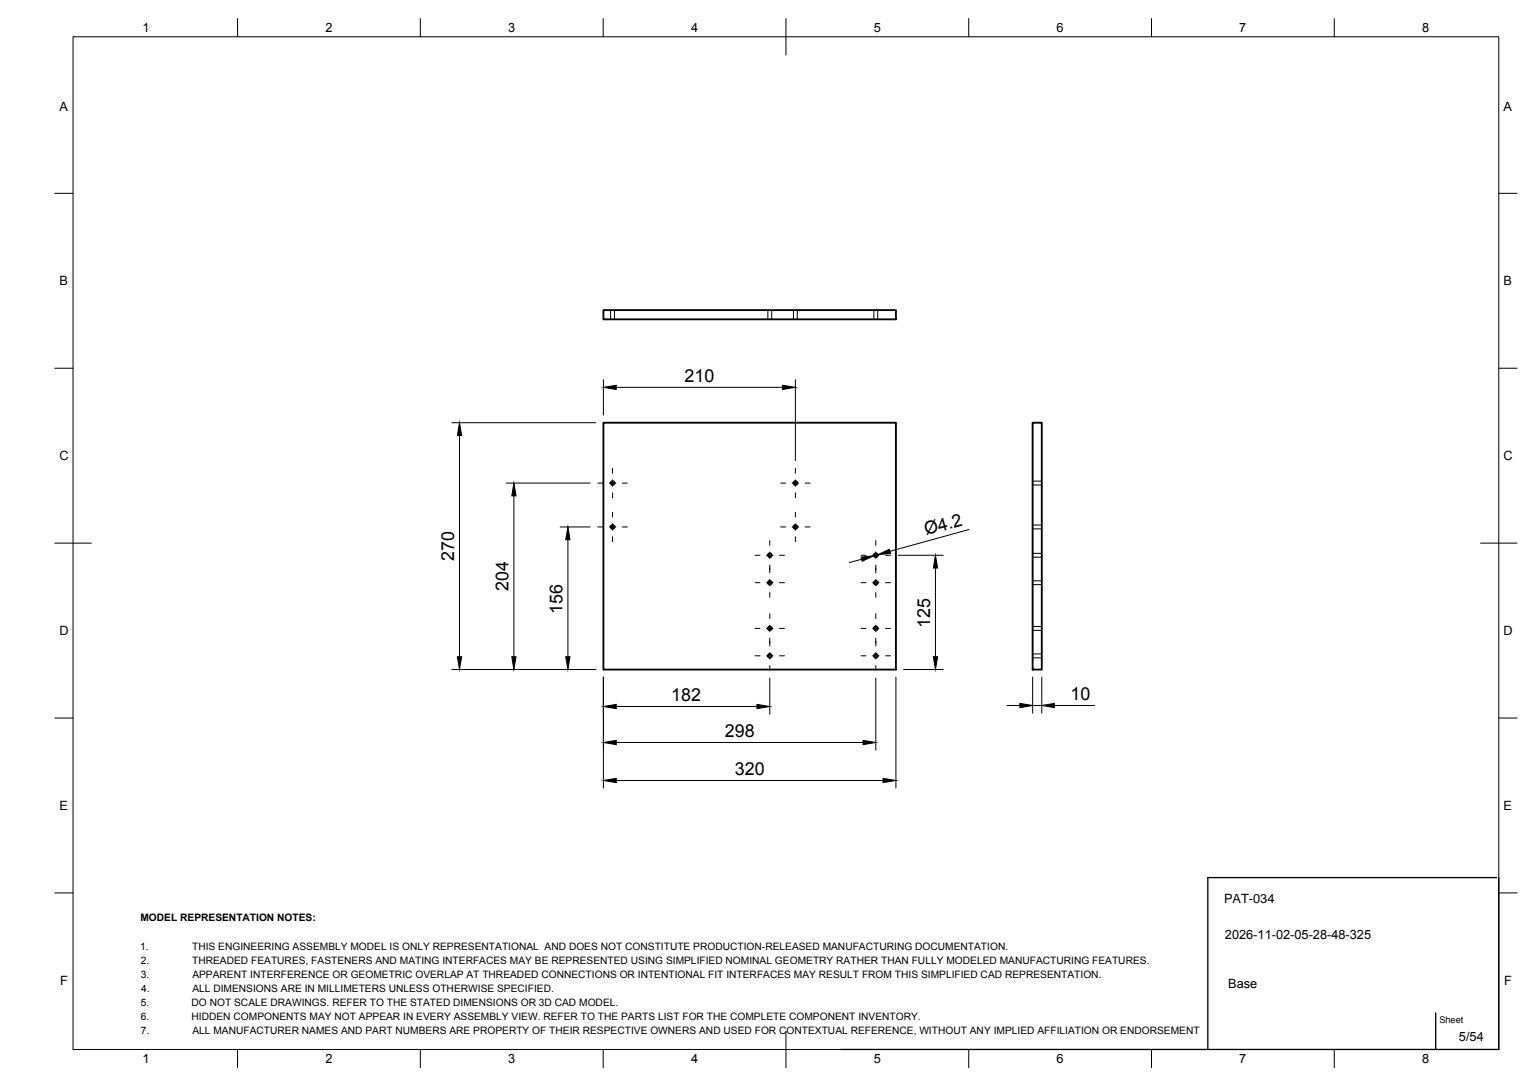
ISO-10303-21;
HEADER;
/* Generated by software containing ST-Developer
 * from STEP Tools, Inc. (www.steptools.com) 
 */

FILE_DESCRIPTION(
/* description */ ('Fatigue rig crank-slider'),
/* implementation_level */ '2;1');

FILE_NAME(
/* name */ 'Base.step',
/* time_stamp */ '2026-10-28T03:24:50-07:00',
/* author */ (''),
/* organization */ (''),
/* preprocessor_version */ 'ST-DEVELOPER v20.2',
/* originating_system */ 'Autodesk Translation Framework v15.17.0.0',
/* authorisation */ '');

FILE_SCHEMA (('AUTOMOTIVE_DESIGN { 1 0 10303 214 3 1 1 }'));
ENDSEC;

DATA;
#10=MECHANICAL_DESIGN_GEOMETRIC_PRESENTATION_REPRESENTATION('',(#587),#16911);
#487=SHAPE_REPRESENTATION_RELATIONSHIP('SRR','None',#17126,#537);
#537=ADVANCED_BREP_SHAPE_REPRESENTATION('',(#646),#16855);
#587=STYLED_ITEM('',(#17466),#646);
#646=MANIFOLD_SOLID_BREP('Body1',#8878);
#700=FACE_BOUND('',#1757,.T.);
#701=FACE_BOUND('',#1758,.T.);
#702=FACE_BOUND('',#1759,.T.);
#703=FACE_BOUND('',#1760,.T.);
#704=FACE_BOUND('',#1761,.T.);
#705=FACE_BOUND('',#1762,.T.);
#706=FACE_BOUND('',#1763,.T.);
#707=FACE_BOUND('',#1764,.T.);
#708=FACE_BOUND('',#1765,.T.);
#709=FACE_BOUND('',#1766,.T.);
#710=FACE_BOUND('',#1767,.T.);
#711=FACE_BOUND('',#1768,.T.);
#712=FACE_BOUND('',#1770,.T.);
#713=FACE_BOUND('',#1771,.T.);
#714=FACE_BOUND('',#1772,.T.);
#715=FACE_BOUND('',#1773,.T.);
#716=FACE_BOUND('',#1774,.T.);
#717=FACE_BOUND('',#1775,.T.);
#718=FACE_BOUND('',#1776,.T.);
#719=FACE_BOUND('',#1777,.T.);
#720=FACE_BOUND('',#1778,.T.);
#721=FACE_BOUND('',#1779,.T.);
#722=FACE_BOUND('',#1780,.T.);
#723=FACE_BOUND('',#1781,.T.);
#897=PLANE('',#9532);
#898=PLANE('',#9533);
#899=PLANE('',#9534);
#900=PLANE('',#9535);
#901=PLANE('',#9536);
#902=PLANE('',#9537);
#1217=FACE_OUTER_BOUND('',#1740,.T.);
#1218=FACE_OUTER_BOUND('',#1741,.T.);
#1219=FACE_OUTER_BOUND('',#1742,.T.);
#1220=FACE_OUTER_BOUND('',#1743,.T.);
#1221=FACE_OUTER_BOUND('',#1744,.T.);
#1222=FACE_OUTER_BOUND('',#1745,.T.);
#1223=FACE_OUTER_BOUND('',#1746,.T.);
#1224=FACE_OUTER_BOUND('',#1747,.T.);
#1225=FACE_OUTER_BOUND('',#1748,.T.);
#1226=FACE_OUTER_BOUND('',#1749,.T.);
#1227=FACE_OUTER_BOUND('',#1750,.T.);
#1228=FACE_OUTER_BOUND('',#1751,.T.);
#1229=FACE_OUTER_BOUND('',#1752,.T.);
#1230=FACE_OUTER_BOUND('',#1753,.T.);
#1231=FACE_OUTER_BOUND('',#1754,.T.);
#1232=FACE_OUTER_BOUND('',#1755,.T.);
#1233=FACE_OUTER_BOUND('',#1756,.T.);
#1234=FACE_OUTER_BOUND('',#1769,.T.);
#1740=EDGE_LOOP('',(#5996,#5997,#5998,#5999));
#1741=EDGE_LOOP('',(#6000,#6001,#6002,#6003));
#1742=EDGE_LOOP('',(#6004,#6005,#6006,#6007));
#1743=EDGE_LOOP('',(#6008,#6009,#6010,#6011));
#1744=EDGE_LOOP('',(#6012,#6013,#6014,#6015));
#1745=EDGE_LOOP('',(#6016,#6017,#6018,#6019));
#1746=EDGE_LOOP('',(#6020,#6021,#6022,#6023));
#1747=EDGE_LOOP('',(#6024,#6025,#6026,#6027));
#1748=EDGE_LOOP('',(#6028,#6029,#6030,#6031));
#1749=EDGE_LOOP('',(#6032,#6033,#6034,#6035));
#1750=EDGE_LOOP('',(#6036,#6037,#6038,#6039));
#1751=EDGE_LOOP('',(#6040,#6041,#6042,#6043));
#1752=EDGE_LOOP('',(#6044,#6045,#6046,#6047));
#1753=EDGE_LOOP('',(#6048,#6049,#6050,#6051));
#1754=EDGE_LOOP('',(#6052,#6053,#6054,#6055));
#1755=EDGE_LOOP('',(#6056,#6057,#6058,#6059));
#1756=EDGE_LOOP('',(#6060,#6061,#6062,#6063));
#1757=EDGE_LOOP('',(#6064));
#1758=EDGE_LOOP('',(#6065));
#1759=EDGE_LOOP('',(#6066));
#1760=EDGE_LOOP('',(#6067));
#1761=EDGE_LOOP('',(#6068));
#1762=EDGE_LOOP('',(#6069));
#1763=EDGE_LOOP('',(#6070));
#1764=EDGE_LOOP('',(#6071));
#1765=EDGE_LOOP('',(#6072));
#1766=EDGE_LOOP('',(#6073));
#1767=EDGE_LOOP('',(#6074));
#1768=EDGE_LOOP('',(#6075));
#1769=EDGE_LOOP('',(#6076,#6077,#6078,#6079));
#1770=EDGE_LOOP('',(#6080));
#1771=EDGE_LOOP('',(#6081));
#1772=EDGE_LOOP('',(#6082));
#1773=EDGE_LOOP('',(#6083));
#1774=EDGE_LOOP('',(#6084));
#1775=EDGE_LOOP('',(#6085));
#1776=EDGE_LOOP('',(#6086));
#1777=EDGE_LOOP('',(#6087));
#1778=EDGE_LOOP('',(#6088));
#1779=EDGE_LOOP('',(#6089));
#1780=EDGE_LOOP('',(#6090));
#1781=EDGE_LOOP('',(#6091));
#2460=LINE('',#13365,#3106);
#2461=LINE('',#13371,#3107);
#2462=LINE('',#13377,#3108);
#2463=LINE('',#13383,#3109);
#2464=LINE('',#13389,#3110);
#2465=LINE('',#13395,#3111);
#2466=LINE('',#13401,#3112);
#2467=LINE('',#13407,#3113);
#2468=LINE('',#13413,#3114);
#2469=LINE('',#13419,#3115);
#2470=LINE('',#13425,#3116);
#2471=LINE('',#13431,#3117);
#2472=LINE('',#13436,#3118);
#2473=LINE('',#13438,#3119);
#2474=LINE('',#13440,#3120);
#2475=LINE('',#13441,#3121);
#2476=LINE('',#13444,#3122);
#2477=LINE('',#13446,#3123);
#2478=LINE('',#13447,#3124);
#2479=LINE('',#13450,#3125);
#2480=LINE('',#13452,#3126);
#2481=LINE('',#13453,#3127);
#2482=LINE('',#13455,#3128);
#2483=LINE('',#13456,#3129);
#3106=VECTOR('',#10576,0.210000000000001);
#3107=VECTOR('',#10583,0.21);
#3108=VECTOR('',#10590,0.21);
#3109=VECTOR('',#10597,0.210000000000001);
#3110=VECTOR('',#10604,0.21);
#3111=VECTOR('',#10611,0.21);
#3112=VECTOR('',#10618,0.21);
#3113=VECTOR('',#10625,0.21);
#3114=VECTOR('',#10632,0.21);
#3115=VECTOR('',#10639,0.21);
#3116=VECTOR('',#10646,0.21);
#3117=VECTOR('',#10653,0.21);
#3118=VECTOR('',#10658,1.);
#3119=VECTOR('',#10659,1.);
#3120=VECTOR('',#10660,1.);
#3121=VECTOR('',#10661,1.);
#3122=VECTOR('',#10664,1.);
#3123=VECTOR('',#10665,1.);
#3124=VECTOR('',#10666,1.);
#3125=VECTOR('',#10669,1.);
#3126=VECTOR('',#10670,1.);
#3127=VECTOR('',#10671,1.);
#3128=VECTOR('',#10674,1.);
#3129=VECTOR('',#10675,1.);
#3752=CIRCLE('',#9497,0.210000000000001);
#3753=CIRCLE('',#9498,0.210000000000001);
#3754=CIRCLE('',#9500,0.21);
#3755=CIRCLE('',#9501,0.21);
#3756=CIRCLE('',#9503,0.21);
#3757=CIRCLE('',#9504,0.21);
#3758=CIRCLE('',#9506,0.210000000000001);
#3759=CIRCLE('',#9507,0.210000000000001);
#3760=CIRCLE('',#9509,0.21);
#3761=CIRCLE('',#9510,0.21);
#3762=CIRCLE('',#9512,0.21);
#3763=CIRCLE('',#9513,0.21);
#3764=CIRCLE('',#9515,0.21);
#3765=CIRCLE('',#9516,0.21);
#3766=CIRCLE('',#9518,0.21);
#3767=CIRCLE('',#9519,0.21);
#3768=CIRCLE('',#9521,0.21);
#3769=CIRCLE('',#9522,0.21);
#3770=CIRCLE('',#9524,0.21);
#3771=CIRCLE('',#9525,0.21);
#3772=CIRCLE('',#9527,0.21);
#3773=CIRCLE('',#9528,0.21);
#3774=CIRCLE('',#9530,0.21);
#3775=CIRCLE('',#9531,0.21);
#4152=VERTEX_POINT('',#13362);
#4153=VERTEX_POINT('',#13364);
#4154=VERTEX_POINT('',#13368);
#4155=VERTEX_POINT('',#13370);
#4156=VERTEX_POINT('',#13374);
#4157=VERTEX_POINT('',#13376);
#4158=VERTEX_POINT('',#13380);
#4159=VERTEX_POINT('',#13382);
#4160=VERTEX_POINT('',#13386);
#4161=VERTEX_POINT('',#13388);
#4162=VERTEX_POINT('',#13392);
#4163=VERTEX_POINT('',#13394);
#4164=VERTEX_POINT('',#13398);
#4165=VERTEX_POINT('',#13400);
#4166=VERTEX_POINT('',#13404);
#4167=VERTEX_POINT('',#13406);
#4168=VERTEX_POINT('',#13410);
#4169=VERTEX_POINT('',#13412);
#4170=VERTEX_POINT('',#13416);
#4171=VERTEX_POINT('',#13418);
#4172=VERTEX_POINT('',#13422);
#4173=VERTEX_POINT('',#13424);
#4174=VERTEX_POINT('',#13428);
#4175=VERTEX_POINT('',#13430);
#4176=VERTEX_POINT('',#13434);
#4177=VERTEX_POINT('',#13435);
#4178=VERTEX_POINT('',#13437);
#4179=VERTEX_POINT('',#13439);
#4180=VERTEX_POINT('',#13443);
#4181=VERTEX_POINT('',#13445);
#4182=VERTEX_POINT('',#13449);
#4183=VERTEX_POINT('',#13451);
#4896=EDGE_CURVE('',#4152,#4152,#3752,.T.);
#4897=EDGE_CURVE('',#4152,#4153,#2460,.T.);
#4898=EDGE_CURVE('',#4153,#4153,#3753,.T.);
#4899=EDGE_CURVE('',#4154,#4154,#3754,.T.);
#4900=EDGE_CURVE('',#4154,#4155,#2461,.T.);
#4901=EDGE_CURVE('',#4155,#4155,#3755,.T.);
#4902=EDGE_CURVE('',#4156,#4156,#3756,.T.);
#4903=EDGE_CURVE('',#4156,#4157,#2462,.T.);
#4904=EDGE_CURVE('',#4157,#4157,#3757,.T.);
#4905=EDGE_CURVE('',#4158,#4158,#3758,.T.);
#4906=EDGE_CURVE('',#4158,#4159,#2463,.T.);
#4907=EDGE_CURVE('',#4159,#4159,#3759,.T.);
#4908=EDGE_CURVE('',#4160,#4160,#3760,.T.);
#4909=EDGE_CURVE('',#4160,#4161,#2464,.T.);
#4910=EDGE_CURVE('',#4161,#4161,#3761,.T.);
#4911=EDGE_CURVE('',#4162,#4162,#3762,.T.);
#4912=EDGE_CURVE('',#4162,#4163,#2465,.T.);
#4913=EDGE_CURVE('',#4163,#4163,#3763,.T.);
#4914=EDGE_CURVE('',#4164,#4164,#3764,.T.);
#4915=EDGE_CURVE('',#4164,#4165,#2466,.T.);
#4916=EDGE_CURVE('',#4165,#4165,#3765,.T.);
#4917=EDGE_CURVE('',#4166,#4166,#3766,.T.);
#4918=EDGE_CURVE('',#4166,#4167,#2467,.T.);
#4919=EDGE_CURVE('',#4167,#4167,#3767,.T.);
#4920=EDGE_CURVE('',#4168,#4168,#3768,.T.);
#4921=EDGE_CURVE('',#4168,#4169,#2468,.T.);
#4922=EDGE_CURVE('',#4169,#4169,#3769,.T.);
#4923=EDGE_CURVE('',#4170,#4170,#3770,.T.);
#4924=EDGE_CURVE('',#4170,#4171,#2469,.T.);
#4925=EDGE_CURVE('',#4171,#4171,#3771,.T.);
#4926=EDGE_CURVE('',#4172,#4172,#3772,.T.);
#4927=EDGE_CURVE('',#4172,#4173,#2470,.T.);
#4928=EDGE_CURVE('',#4173,#4173,#3773,.T.);
#4929=EDGE_CURVE('',#4174,#4174,#3774,.T.);
#4930=EDGE_CURVE('',#4174,#4175,#2471,.T.);
#4931=EDGE_CURVE('',#4175,#4175,#3775,.T.);
#4932=EDGE_CURVE('',#4176,#4177,#2472,.T.);
#4933=EDGE_CURVE('',#4177,#4178,#2473,.T.);
#4934=EDGE_CURVE('',#4179,#4178,#2474,.T.);
#4935=EDGE_CURVE('',#4176,#4179,#2475,.T.);
#4936=EDGE_CURVE('',#4180,#4176,#2476,.T.);
#4937=EDGE_CURVE('',#4181,#4179,#2477,.T.);
#4938=EDGE_CURVE('',#4180,#4181,#2478,.T.);
#4939=EDGE_CURVE('',#4182,#4180,#2479,.T.);
#4940=EDGE_CURVE('',#4183,#4181,#2480,.T.);
#4941=EDGE_CURVE('',#4182,#4183,#2481,.T.);
#4942=EDGE_CURVE('',#4177,#4182,#2482,.T.);
#4943=EDGE_CURVE('',#4178,#4183,#2483,.T.);
#5996=ORIENTED_EDGE('',*,*,#4896,.F.);
#5997=ORIENTED_EDGE('',*,*,#4897,.T.);
#5998=ORIENTED_EDGE('',*,*,#4898,.F.);
#5999=ORIENTED_EDGE('',*,*,#4897,.F.);
#6000=ORIENTED_EDGE('',*,*,#4899,.F.);
#6001=ORIENTED_EDGE('',*,*,#4900,.T.);
#6002=ORIENTED_EDGE('',*,*,#4901,.F.);
#6003=ORIENTED_EDGE('',*,*,#4900,.F.);
#6004=ORIENTED_EDGE('',*,*,#4902,.F.);
#6005=ORIENTED_EDGE('',*,*,#4903,.T.);
#6006=ORIENTED_EDGE('',*,*,#4904,.F.);
#6007=ORIENTED_EDGE('',*,*,#4903,.F.);
#6008=ORIENTED_EDGE('',*,*,#4905,.F.);
#6009=ORIENTED_EDGE('',*,*,#4906,.T.);
#6010=ORIENTED_EDGE('',*,*,#4907,.F.);
#6011=ORIENTED_EDGE('',*,*,#4906,.F.);
#6012=ORIENTED_EDGE('',*,*,#4908,.F.);
#6013=ORIENTED_EDGE('',*,*,#4909,.T.);
#6014=ORIENTED_EDGE('',*,*,#4910,.F.);
#6015=ORIENTED_EDGE('',*,*,#4909,.F.);
#6016=ORIENTED_EDGE('',*,*,#4911,.F.);
#6017=ORIENTED_EDGE('',*,*,#4912,.T.);
#6018=ORIENTED_EDGE('',*,*,#4913,.F.);
#6019=ORIENTED_EDGE('',*,*,#4912,.F.);
#6020=ORIENTED_EDGE('',*,*,#4914,.F.);
#6021=ORIENTED_EDGE('',*,*,#4915,.T.);
#6022=ORIENTED_EDGE('',*,*,#4916,.F.);
#6023=ORIENTED_EDGE('',*,*,#4915,.F.);
#6024=ORIENTED_EDGE('',*,*,#4917,.F.);
#6025=ORIENTED_EDGE('',*,*,#4918,.T.);
#6026=ORIENTED_EDGE('',*,*,#4919,.F.);
#6027=ORIENTED_EDGE('',*,*,#4918,.F.);
#6028=ORIENTED_EDGE('',*,*,#4920,.F.);
#6029=ORIENTED_EDGE('',*,*,#4921,.T.);
#6030=ORIENTED_EDGE('',*,*,#4922,.F.);
#6031=ORIENTED_EDGE('',*,*,#4921,.F.);
#6032=ORIENTED_EDGE('',*,*,#4923,.F.);
#6033=ORIENTED_EDGE('',*,*,#4924,.T.);
#6034=ORIENTED_EDGE('',*,*,#4925,.F.);
#6035=ORIENTED_EDGE('',*,*,#4924,.F.);
#6036=ORIENTED_EDGE('',*,*,#4926,.F.);
#6037=ORIENTED_EDGE('',*,*,#4927,.T.);
#6038=ORIENTED_EDGE('',*,*,#4928,.F.);
#6039=ORIENTED_EDGE('',*,*,#4927,.F.);
#6040=ORIENTED_EDGE('',*,*,#4929,.F.);
#6041=ORIENTED_EDGE('',*,*,#4930,.T.);
#6042=ORIENTED_EDGE('',*,*,#4931,.F.);
#6043=ORIENTED_EDGE('',*,*,#4930,.F.);
#6044=ORIENTED_EDGE('',*,*,#4932,.T.);
#6045=ORIENTED_EDGE('',*,*,#4933,.T.);
#6046=ORIENTED_EDGE('',*,*,#4934,.F.);
#6047=ORIENTED_EDGE('',*,*,#4935,.F.);
#6048=ORIENTED_EDGE('',*,*,#4936,.T.);
#6049=ORIENTED_EDGE('',*,*,#4935,.T.);
#6050=ORIENTED_EDGE('',*,*,#4937,.F.);
#6051=ORIENTED_EDGE('',*,*,#4938,.F.);
#6052=ORIENTED_EDGE('',*,*,#4939,.T.);
#6053=ORIENTED_EDGE('',*,*,#4938,.T.);
#6054=ORIENTED_EDGE('',*,*,#4940,.F.);
#6055=ORIENTED_EDGE('',*,*,#4941,.F.);
#6056=ORIENTED_EDGE('',*,*,#4942,.T.);
#6057=ORIENTED_EDGE('',*,*,#4941,.T.);
#6058=ORIENTED_EDGE('',*,*,#4943,.F.);
#6059=ORIENTED_EDGE('',*,*,#4933,.F.);
#6060=ORIENTED_EDGE('',*,*,#4943,.T.);
#6061=ORIENTED_EDGE('',*,*,#4940,.T.);
#6062=ORIENTED_EDGE('',*,*,#4937,.T.);
#6063=ORIENTED_EDGE('',*,*,#4934,.T.);
#6064=ORIENTED_EDGE('',*,*,#4910,.T.);
#6065=ORIENTED_EDGE('',*,*,#4913,.T.);
#6066=ORIENTED_EDGE('',*,*,#4916,.T.);
#6067=ORIENTED_EDGE('',*,*,#4919,.T.);
#6068=ORIENTED_EDGE('',*,*,#4922,.T.);
#6069=ORIENTED_EDGE('',*,*,#4925,.T.);
#6070=ORIENTED_EDGE('',*,*,#4928,.T.);
#6071=ORIENTED_EDGE('',*,*,#4931,.T.);
#6072=ORIENTED_EDGE('',*,*,#4907,.T.);
#6073=ORIENTED_EDGE('',*,*,#4904,.T.);
#6074=ORIENTED_EDGE('',*,*,#4901,.T.);
#6075=ORIENTED_EDGE('',*,*,#4898,.T.);
#6076=ORIENTED_EDGE('',*,*,#4942,.F.);
#6077=ORIENTED_EDGE('',*,*,#4932,.F.);
#6078=ORIENTED_EDGE('',*,*,#4936,.F.);
#6079=ORIENTED_EDGE('',*,*,#4939,.F.);
#6080=ORIENTED_EDGE('',*,*,#4908,.T.);
#6081=ORIENTED_EDGE('',*,*,#4911,.T.);
#6082=ORIENTED_EDGE('',*,*,#4914,.T.);
#6083=ORIENTED_EDGE('',*,*,#4917,.T.);
#6084=ORIENTED_EDGE('',*,*,#4920,.T.);
#6085=ORIENTED_EDGE('',*,*,#4923,.T.);
#6086=ORIENTED_EDGE('',*,*,#4926,.T.);
#6087=ORIENTED_EDGE('',*,*,#4929,.T.);
#6088=ORIENTED_EDGE('',*,*,#4905,.T.);
#6089=ORIENTED_EDGE('',*,*,#4902,.T.);
#6090=ORIENTED_EDGE('',*,*,#4899,.T.);
#6091=ORIENTED_EDGE('',*,*,#4896,.T.);
#8196=CYLINDRICAL_SURFACE('',#9496,0.210000000000001);
#8197=CYLINDRICAL_SURFACE('',#9499,0.21);
#8198=CYLINDRICAL_SURFACE('',#9502,0.21);
#8199=CYLINDRICAL_SURFACE('',#9505,0.210000000000001);
#8200=CYLINDRICAL_SURFACE('',#9508,0.21);
#8201=CYLINDRICAL_SURFACE('',#9511,0.21);
#8202=CYLINDRICAL_SURFACE('',#9514,0.21);
#8203=CYLINDRICAL_SURFACE('',#9517,0.21);
#8204=CYLINDRICAL_SURFACE('',#9520,0.21);
#8205=CYLINDRICAL_SURFACE('',#9523,0.21);
#8206=CYLINDRICAL_SURFACE('',#9526,0.21);
#8207=CYLINDRICAL_SURFACE('',#9529,0.21);
#8355=ADVANCED_FACE('',(#1217),#8196,.F.);
#8356=ADVANCED_FACE('',(#1218),#8197,.F.);
#8357=ADVANCED_FACE('',(#1219),#8198,.F.);
#8358=ADVANCED_FACE('',(#1220),#8199,.F.);
#8359=ADVANCED_FACE('',(#1221),#8200,.F.);
#8360=ADVANCED_FACE('',(#1222),#8201,.F.);
#8361=ADVANCED_FACE('',(#1223),#8202,.F.);
#8362=ADVANCED_FACE('',(#1224),#8203,.F.);
#8363=ADVANCED_FACE('',(#1225),#8204,.F.);
#8364=ADVANCED_FACE('',(#1226),#8205,.F.);
#8365=ADVANCED_FACE('',(#1227),#8206,.F.);
#8366=ADVANCED_FACE('',(#1228),#8207,.F.);
#8367=ADVANCED_FACE('',(#1229),#897,.T.);
#8368=ADVANCED_FACE('',(#1230),#898,.T.);
#8369=ADVANCED_FACE('',(#1231),#899,.T.);
#8370=ADVANCED_FACE('',(#1232),#900,.T.);
#8371=ADVANCED_FACE('',(#1233,#700,#701,#702,#703,#704,#705,#706,#707,#708,
#709,#710,#711),#901,.T.);
#8372=ADVANCED_FACE('',(#1234,#712,#713,#714,#715,#716,#717,#718,#719,#720,
#721,#722,#723),#902,.F.);
#8878=CLOSED_SHELL('',(#8355,#8356,#8357,#8358,#8359,#8360,#8361,#8362,
#8363,#8364,#8365,#8366,#8367,#8368,#8369,#8370,#8371,#8372));
#9495=AXIS2_PLACEMENT_3D('',#13360,#10570,#10571);
#9496=AXIS2_PLACEMENT_3D('',#13361,#10572,#10573);
#9497=AXIS2_PLACEMENT_3D('',#13363,#10574,#10575);
#9498=AXIS2_PLACEMENT_3D('',#13366,#10577,#10578);
#9499=AXIS2_PLACEMENT_3D('',#13367,#10579,#10580);
#9500=AXIS2_PLACEMENT_3D('',#13369,#10581,#10582);
#9501=AXIS2_PLACEMENT_3D('',#13372,#10584,#10585);
#9502=AXIS2_PLACEMENT_3D('',#13373,#10586,#10587);
#9503=AXIS2_PLACEMENT_3D('',#13375,#10588,#10589);
#9504=AXIS2_PLACEMENT_3D('',#13378,#10591,#10592);
#9505=AXIS2_PLACEMENT_3D('',#13379,#10593,#10594);
#9506=AXIS2_PLACEMENT_3D('',#13381,#10595,#10596);
#9507=AXIS2_PLACEMENT_3D('',#13384,#10598,#10599);
#9508=AXIS2_PLACEMENT_3D('',#13385,#10600,#10601);
#9509=AXIS2_PLACEMENT_3D('',#13387,#10602,#10603);
#9510=AXIS2_PLACEMENT_3D('',#13390,#10605,#10606);
#9511=AXIS2_PLACEMENT_3D('',#13391,#10607,#10608);
#9512=AXIS2_PLACEMENT_3D('',#13393,#10609,#10610);
#9513=AXIS2_PLACEMENT_3D('',#13396,#10612,#10613);
#9514=AXIS2_PLACEMENT_3D('',#13397,#10614,#10615);
#9515=AXIS2_PLACEMENT_3D('',#13399,#10616,#10617);
#9516=AXIS2_PLACEMENT_3D('',#13402,#10619,#10620);
#9517=AXIS2_PLACEMENT_3D('',#13403,#10621,#10622);
#9518=AXIS2_PLACEMENT_3D('',#13405,#10623,#10624);
#9519=AXIS2_PLACEMENT_3D('',#13408,#10626,#10627);
#9520=AXIS2_PLACEMENT_3D('',#13409,#10628,#10629);
#9521=AXIS2_PLACEMENT_3D('',#13411,#10630,#10631);
#9522=AXIS2_PLACEMENT_3D('',#13414,#10633,#10634);
#9523=AXIS2_PLACEMENT_3D('',#13415,#10635,#10636);
#9524=AXIS2_PLACEMENT_3D('',#13417,#10637,#10638);
#9525=AXIS2_PLACEMENT_3D('',#13420,#10640,#10641);
#9526=AXIS2_PLACEMENT_3D('',#13421,#10642,#10643);
#9527=AXIS2_PLACEMENT_3D('',#13423,#10644,#10645);
#9528=AXIS2_PLACEMENT_3D('',#13426,#10647,#10648);
#9529=AXIS2_PLACEMENT_3D('',#13427,#10649,#10650);
#9530=AXIS2_PLACEMENT_3D('',#13429,#10651,#10652);
#9531=AXIS2_PLACEMENT_3D('',#13432,#10654,#10655);
#9532=AXIS2_PLACEMENT_3D('',#13433,#10656,#10657);
#9533=AXIS2_PLACEMENT_3D('',#13442,#10662,#10663);
#9534=AXIS2_PLACEMENT_3D('',#13448,#10667,#10668);
#9535=AXIS2_PLACEMENT_3D('',#13454,#10672,#10673);
#9536=AXIS2_PLACEMENT_3D('',#13457,#10676,#10677);
#9537=AXIS2_PLACEMENT_3D('',#13458,#10678,#10679);
#10570=DIRECTION('axis',(0.,0.,1.));
#10571=DIRECTION('refdir',(1.,0.,0.));
#10572=DIRECTION('center_axis',(0.,0.,1.));
#10573=DIRECTION('ref_axis',(1.,0.,0.));
#10574=DIRECTION('center_axis',(0.,0.,1.));
#10575=DIRECTION('ref_axis',(1.,0.,0.));
#10576=DIRECTION('',(0.,0.,1.));
#10577=DIRECTION('center_axis',(0.,0.,-1.));
#10578=DIRECTION('ref_axis',(1.,0.,0.));
#10579=DIRECTION('center_axis',(0.,0.,1.));
#10580=DIRECTION('ref_axis',(1.,0.,0.));
#10581=DIRECTION('center_axis',(0.,0.,1.));
#10582=DIRECTION('ref_axis',(1.,0.,0.));
#10583=DIRECTION('',(0.,0.,1.));
#10584=DIRECTION('center_axis',(0.,0.,-1.));
#10585=DIRECTION('ref_axis',(1.,0.,0.));
#10586=DIRECTION('center_axis',(0.,0.,1.));
#10587=DIRECTION('ref_axis',(1.,0.,0.));
#10588=DIRECTION('center_axis',(0.,0.,1.));
#10589=DIRECTION('ref_axis',(1.,0.,0.));
#10590=DIRECTION('',(0.,0.,1.));
#10591=DIRECTION('center_axis',(0.,0.,-1.));
#10592=DIRECTION('ref_axis',(1.,0.,0.));
#10593=DIRECTION('center_axis',(0.,0.,1.));
#10594=DIRECTION('ref_axis',(1.,0.,0.));
#10595=DIRECTION('center_axis',(0.,0.,1.));
#10596=DIRECTION('ref_axis',(1.,0.,0.));
#10597=DIRECTION('',(0.,0.,1.));
#10598=DIRECTION('center_axis',(0.,0.,-1.));
#10599=DIRECTION('ref_axis',(1.,0.,0.));
#10600=DIRECTION('center_axis',(0.,0.,1.));
#10601=DIRECTION('ref_axis',(1.,0.,0.));
#10602=DIRECTION('center_axis',(0.,0.,1.));
#10603=DIRECTION('ref_axis',(1.,0.,0.));
#10604=DIRECTION('',(0.,0.,1.));
#10605=DIRECTION('center_axis',(0.,0.,-1.));
#10606=DIRECTION('ref_axis',(1.,0.,0.));
#10607=DIRECTION('center_axis',(0.,0.,1.));
#10608=DIRECTION('ref_axis',(1.,0.,0.));
#10609=DIRECTION('center_axis',(0.,0.,1.));
#10610=DIRECTION('ref_axis',(1.,0.,0.));
#10611=DIRECTION('',(0.,0.,1.));
#10612=DIRECTION('center_axis',(0.,0.,-1.));
#10613=DIRECTION('ref_axis',(1.,0.,0.));
#10614=DIRECTION('center_axis',(0.,0.,1.));
#10615=DIRECTION('ref_axis',(1.,0.,0.));
#10616=DIRECTION('center_axis',(0.,0.,1.));
#10617=DIRECTION('ref_axis',(1.,0.,0.));
#10618=DIRECTION('',(0.,0.,1.));
#10619=DIRECTION('center_axis',(0.,0.,-1.));
#10620=DIRECTION('ref_axis',(1.,0.,0.));
#10621=DIRECTION('center_axis',(0.,0.,1.));
#10622=DIRECTION('ref_axis',(1.,0.,0.));
#10623=DIRECTION('center_axis',(0.,0.,1.));
#10624=DIRECTION('ref_axis',(1.,0.,0.));
#10625=DIRECTION('',(0.,0.,1.));
#10626=DIRECTION('center_axis',(0.,0.,-1.));
#10627=DIRECTION('ref_axis',(1.,0.,0.));
#10628=DIRECTION('center_axis',(0.,0.,1.));
#10629=DIRECTION('ref_axis',(1.,0.,0.));
#10630=DIRECTION('center_axis',(0.,0.,1.));
#10631=DIRECTION('ref_axis',(1.,0.,0.));
#10632=DIRECTION('',(0.,0.,1.));
#10633=DIRECTION('center_axis',(0.,0.,-1.));
#10634=DIRECTION('ref_axis',(1.,0.,0.));
#10635=DIRECTION('center_axis',(0.,0.,1.));
#10636=DIRECTION('ref_axis',(1.,0.,0.));
#10637=DIRECTION('center_axis',(0.,0.,1.));
#10638=DIRECTION('ref_axis',(1.,0.,0.));
#10639=DIRECTION('',(0.,0.,1.));
#10640=DIRECTION('center_axis',(0.,0.,-1.));
#10641=DIRECTION('ref_axis',(1.,0.,0.));
#10642=DIRECTION('center_axis',(0.,0.,1.));
#10643=DIRECTION('ref_axis',(1.,0.,0.));
#10644=DIRECTION('center_axis',(0.,0.,1.));
#10645=DIRECTION('ref_axis',(1.,0.,0.));
#10646=DIRECTION('',(0.,0.,1.));
#10647=DIRECTION('center_axis',(0.,0.,-1.));
#10648=DIRECTION('ref_axis',(1.,0.,0.));
#10649=DIRECTION('center_axis',(0.,0.,1.));
#10650=DIRECTION('ref_axis',(1.,0.,0.));
#10651=DIRECTION('center_axis',(0.,0.,1.));
#10652=DIRECTION('ref_axis',(1.,0.,0.));
#10653=DIRECTION('',(0.,0.,1.));
#10654=DIRECTION('center_axis',(0.,0.,-1.));
#10655=DIRECTION('ref_axis',(1.,0.,0.));
#10656=DIRECTION('center_axis',(0.,1.,0.));
#10657=DIRECTION('ref_axis',(-1.,0.,0.));
#10658=DIRECTION('',(-1.,0.,0.));
#10659=DIRECTION('',(0.,0.,1.));
#10660=DIRECTION('',(-1.,0.,0.));
#10661=DIRECTION('',(0.,0.,1.));
#10662=DIRECTION('center_axis',(1.,0.,0.));
#10663=DIRECTION('ref_axis',(0.,1.,0.));
#10664=DIRECTION('',(0.,1.,0.));
#10665=DIRECTION('',(0.,1.,0.));
#10666=DIRECTION('',(0.,0.,1.));
#10667=DIRECTION('center_axis',(0.,-1.,0.));
#10668=DIRECTION('ref_axis',(1.,0.,0.));
#10669=DIRECTION('',(1.,0.,0.));
#10670=DIRECTION('',(1.,0.,0.));
#10671=DIRECTION('',(0.,0.,1.));
#10672=DIRECTION('center_axis',(-1.,0.,0.));
#10673=DIRECTION('ref_axis',(0.,-1.,0.));
#10674=DIRECTION('',(0.,-1.,0.));
#10675=DIRECTION('',(0.,-1.,0.));
#10676=DIRECTION('center_axis',(0.,0.,1.));
#10677=DIRECTION('ref_axis',(1.,0.,0.));
#10678=DIRECTION('center_axis',(0.,0.,1.));
#10679=DIRECTION('ref_axis',(1.,0.,0.));
#13360=CARTESIAN_POINT('',(0.,0.,0.));
#13361=CARTESIAN_POINT('Origin',(23.,-2.4,-0.1));
#13362=CARTESIAN_POINT('',(22.79,-2.4,0.));
#13363=CARTESIAN_POINT('Origin',(23.,-2.4,0.));
#13364=CARTESIAN_POINT('',(22.79,-2.4,1.));
#13365=CARTESIAN_POINT('',(22.79,-2.4,-0.1));
#13366=CARTESIAN_POINT('Origin',(23.,-2.4,1.));
#13367=CARTESIAN_POINT('Origin',(3.,2.4,-0.1));
#13368=CARTESIAN_POINT('',(2.79,2.4,0.));
#13369=CARTESIAN_POINT('Origin',(3.,2.4,0.));
#13370=CARTESIAN_POINT('',(2.79,2.4,1.));
#13371=CARTESIAN_POINT('',(2.79,2.4,-0.1));
#13372=CARTESIAN_POINT('Origin',(3.,2.4,1.));
#13373=CARTESIAN_POINT('Origin',(3.,-2.4,-0.1));
#13374=CARTESIAN_POINT('',(2.79,-2.4,0.));
#13375=CARTESIAN_POINT('Origin',(3.,-2.4,0.));
#13376=CARTESIAN_POINT('',(2.79,-2.4,1.));
#13377=CARTESIAN_POINT('',(2.79,-2.4,-0.1));
#13378=CARTESIAN_POINT('Origin',(3.,-2.4,1.));
#13379=CARTESIAN_POINT('Origin',(23.,2.4,-0.1));
#13380=CARTESIAN_POINT('',(22.79,2.4,0.));
#13381=CARTESIAN_POINT('Origin',(23.,2.4,0.));
#13382=CARTESIAN_POINT('',(22.79,2.4,1.));
#13383=CARTESIAN_POINT('',(22.79,2.4,-0.1));
#13384=CARTESIAN_POINT('Origin',(23.,2.4,1.));
#13385=CARTESIAN_POINT('Origin',(5.8,-8.5,-0.1));
#13386=CARTESIAN_POINT('',(5.59,-8.5,0.));
#13387=CARTESIAN_POINT('Origin',(5.8,-8.5,0.));
#13388=CARTESIAN_POINT('',(5.59,-8.5,1.));
#13389=CARTESIAN_POINT('',(5.59,-8.5,-0.1));
#13390=CARTESIAN_POINT('Origin',(5.8,-8.5,1.));
#13391=CARTESIAN_POINT('Origin',(-5.8,-5.5,-0.1));
#13392=CARTESIAN_POINT('',(-6.01,-5.5,0.));
#13393=CARTESIAN_POINT('Origin',(-5.8,-5.5,0.));
#13394=CARTESIAN_POINT('',(-6.01,-5.5,1.));
#13395=CARTESIAN_POINT('',(-6.01,-5.5,-0.1));
#13396=CARTESIAN_POINT('Origin',(-5.8,-5.5,1.));
#13397=CARTESIAN_POINT('Origin',(-5.8,-8.5,-0.1));
#13398=CARTESIAN_POINT('',(-6.01,-8.5,0.));
#13399=CARTESIAN_POINT('Origin',(-5.8,-8.5,0.));
#13400=CARTESIAN_POINT('',(-6.01,-8.5,1.));
#13401=CARTESIAN_POINT('',(-6.01,-8.5,-0.1));
#13402=CARTESIAN_POINT('Origin',(-5.8,-8.5,1.));
#13403=CARTESIAN_POINT('Origin',(5.8,-5.5,-0.1));
#13404=CARTESIAN_POINT('',(5.59,-5.5,0.));
#13405=CARTESIAN_POINT('Origin',(5.8,-5.5,0.));
#13406=CARTESIAN_POINT('',(5.59,-5.5,1.));
#13407=CARTESIAN_POINT('',(5.59,-5.5,-0.1));
#13408=CARTESIAN_POINT('Origin',(5.8,-5.5,1.));
#13409=CARTESIAN_POINT('Origin',(5.8,-16.5,-0.1));
#13410=CARTESIAN_POINT('',(5.59,-16.5,0.));
#13411=CARTESIAN_POINT('Origin',(5.8,-16.5,0.));
#13412=CARTESIAN_POINT('',(5.59,-16.5,1.));
#13413=CARTESIAN_POINT('',(5.59,-16.5,-0.1));
#13414=CARTESIAN_POINT('Origin',(5.8,-16.5,1.));
#13415=CARTESIAN_POINT('Origin',(-5.8,-13.5,-0.1));
#13416=CARTESIAN_POINT('',(-6.01,-13.5,0.));
#13417=CARTESIAN_POINT('Origin',(-5.8,-13.5,0.));
#13418=CARTESIAN_POINT('',(-6.01,-13.5,1.));
#13419=CARTESIAN_POINT('',(-6.01,-13.5,-0.1));
#13420=CARTESIAN_POINT('Origin',(-5.8,-13.5,1.));
#13421=CARTESIAN_POINT('Origin',(-5.8,-16.5,-0.1));
#13422=CARTESIAN_POINT('',(-6.01,-16.5,0.));
#13423=CARTESIAN_POINT('Origin',(-5.8,-16.5,0.));
#13424=CARTESIAN_POINT('',(-6.01,-16.5,1.));
#13425=CARTESIAN_POINT('',(-6.01,-16.5,-0.1));
#13426=CARTESIAN_POINT('Origin',(-5.8,-16.5,1.));
#13427=CARTESIAN_POINT('Origin',(5.8,-13.5,-0.1));
#13428=CARTESIAN_POINT('',(5.59,-13.5,0.));
#13429=CARTESIAN_POINT('Origin',(5.8,-13.5,0.));
#13430=CARTESIAN_POINT('',(5.59,-13.5,1.));
#13431=CARTESIAN_POINT('',(5.59,-13.5,-0.1));
#13432=CARTESIAN_POINT('Origin',(5.8,-13.5,1.));
#13433=CARTESIAN_POINT('Origin',(24.,9.,0.));
#13434=CARTESIAN_POINT('',(24.,9.,0.));
#13435=CARTESIAN_POINT('',(-8.,9.,0.));
#13436=CARTESIAN_POINT('',(24.,9.,0.));
#13437=CARTESIAN_POINT('',(-8.,9.,1.));
#13438=CARTESIAN_POINT('',(-8.,9.,0.));
#13439=CARTESIAN_POINT('',(24.,9.,1.));
#13440=CARTESIAN_POINT('',(24.,9.,1.));
#13441=CARTESIAN_POINT('',(24.,9.,0.));
#13442=CARTESIAN_POINT('Origin',(24.,-18.,0.));
#13443=CARTESIAN_POINT('',(24.,-18.,0.));
#13444=CARTESIAN_POINT('',(24.,-18.,0.));
#13445=CARTESIAN_POINT('',(24.,-18.,1.));
#13446=CARTESIAN_POINT('',(24.,-18.,1.));
#13447=CARTESIAN_POINT('',(24.,-18.,0.));
#13448=CARTESIAN_POINT('Origin',(-8.,-18.,0.));
#13449=CARTESIAN_POINT('',(-8.,-18.,0.));
#13450=CARTESIAN_POINT('',(-8.,-18.,0.));
#13451=CARTESIAN_POINT('',(-8.,-18.,1.));
#13452=CARTESIAN_POINT('',(-8.,-18.,1.));
#13453=CARTESIAN_POINT('',(-8.,-18.,0.));
#13454=CARTESIAN_POINT('Origin',(-8.,9.,0.));
#13455=CARTESIAN_POINT('',(-8.,9.,0.));
#13456=CARTESIAN_POINT('',(-8.,9.,1.));
#13457=CARTESIAN_POINT('Origin',(8.,-4.5,1.));
#13458=CARTESIAN_POINT('Origin',(8.,-4.5,0.));
#16796=UNCERTAINTY_MEASURE_WITH_UNIT(LENGTH_MEASURE(0.001),#16912,
'DISTANCE_ACCURACY_VALUE',
'Maximum model space distance between geometric entities at asserted c
onnectivities');
#16852=UNCERTAINTY_MEASURE_WITH_UNIT(LENGTH_MEASURE(0.001),#16912,
'DISTANCE_ACCURACY_VALUE',
'Maximum model space distance between geometric entities at asserted c
onnectivities');
#16855=(
GEOMETRIC_REPRESENTATION_CONTEXT(3)
GLOBAL_UNCERTAINTY_ASSIGNED_CONTEXT((#16796))
GLOBAL_UNIT_ASSIGNED_CONTEXT((#16912,#16914,#16915))
REPRESENTATION_CONTEXT('','3D')
);
#16911=(
GEOMETRIC_REPRESENTATION_CONTEXT(3)
GLOBAL_UNCERTAINTY_ASSIGNED_CONTEXT((#16852))
GLOBAL_UNIT_ASSIGNED_CONTEXT((#16912,#16914,#16915))
REPRESENTATION_CONTEXT('','3D')
);
#16912=(
LENGTH_UNIT()
NAMED_UNIT(*)
SI_UNIT(.CENTI.,.METRE.)
);
#16914=(
NAMED_UNIT(*)
PLANE_ANGLE_UNIT()
SI_UNIT($,.RADIAN.)
);
#16915=(
NAMED_UNIT(*)
SI_UNIT($,.STERADIAN.)
SOLID_ANGLE_UNIT()
);
#16918=SHAPE_DEFINITION_REPRESENTATION(#16976,#17126);
#16976=PRODUCT_DEFINITION_SHAPE('',$,#17185);
#17126=SHAPE_REPRESENTATION('',(#9495),#16855);
#17182=PRODUCT_DEFINITION_CONTEXT('part definition',#17358,'design');
#17185=PRODUCT_DEFINITION('Base','Base',#17243,#17182);
#17243=PRODUCT_DEFINITION_FORMATION('',$,#17362);
#17358=APPLICATION_CONTEXT(
'Core Data for Automotive Mechanical Design Process');
#17359=PRODUCT_CONTEXT('part definition',#17358,'mechanical');
#17362=PRODUCT('Base','Base','Base',(#17359));
#17460=COLOUR_RGB('Dark Blue',0.08,0.2,0.34);
#17461=FILL_AREA_STYLE_COLOUR('',#17460);
#17462=FILL_AREA_STYLE('',(#17461));
#17463=SURFACE_STYLE_FILL_AREA(#17462);
#17464=SURFACE_SIDE_STYLE('',(#17463));
#17465=SURFACE_STYLE_USAGE(.BOTH.,#17464);
#17466=PRESENTATION_STYLE_ASSIGNMENT((#17465));
ENDSEC;
END-ISO-10303-21;
